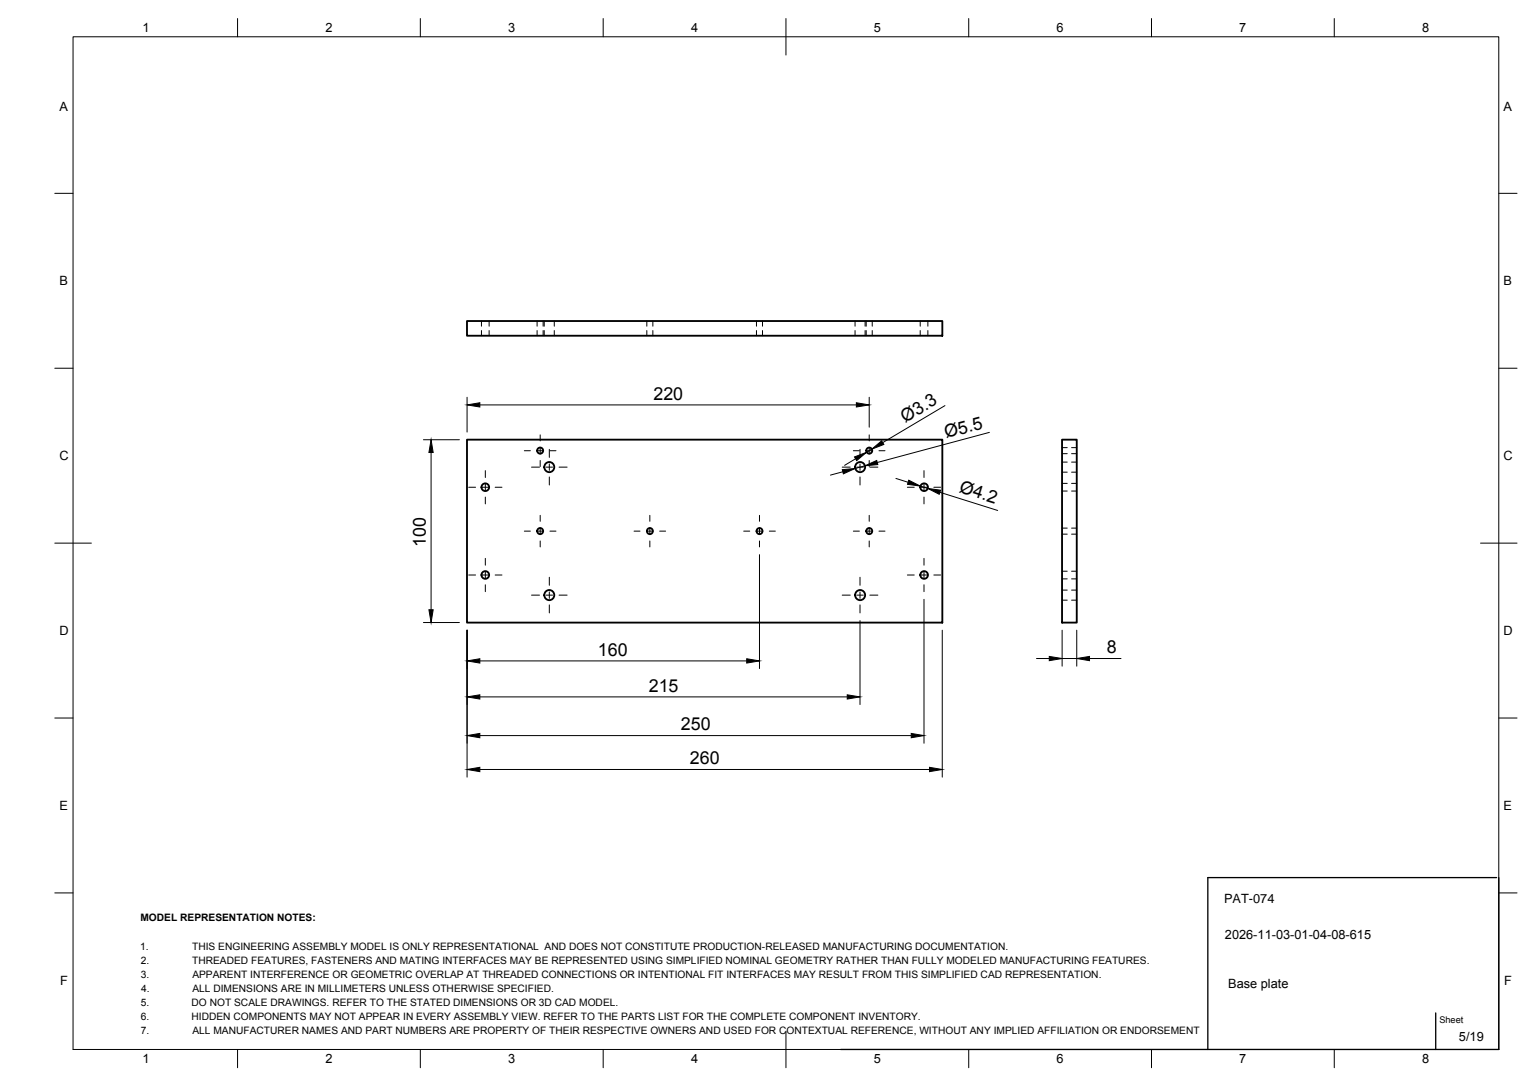
ISO-10303-21;
HEADER;
/* Generated by software containing ST-Developer
 * from STEP Tools, Inc. (www.steptools.com) 
 */

FILE_DESCRIPTION(
/* description */ ('Manual rail carriage with stops'),
/* implementation_level */ '2;1');

FILE_NAME(
/* name */ 'Base plate.step',
/* time_stamp */ '2026-10-27T18:54:27-07:00',
/* author */ (''),
/* organization */ (''),
/* preprocessor_version */ 'ST-DEVELOPER v20.2',
/* originating_system */ 'Autodesk Translation Framework v15.17.0.0',
/* authorisation */ '');

FILE_SCHEMA (('AUTOMOTIVE_DESIGN { 1 0 10303 214 3 1 1 }'));
ENDSEC;

DATA;
#10=MECHANICAL_DESIGN_GEOMETRIC_PRESENTATION_REPRESENTATION('',(#273),#8499);
#237=SHAPE_REPRESENTATION_RELATIONSHIP('SRR','None',#8600,#255);
#255=ADVANCED_BREP_SHAPE_REPRESENTATION('',(#291),#8479);
#273=STYLED_ITEM('',(#8767),#291);
#291=MANIFOLD_SOLID_BREP('Body1',#4941);
#305=FACE_BOUND('',#861,.T.);
#306=FACE_BOUND('',#862,.T.);
#307=FACE_BOUND('',#863,.T.);
#308=FACE_BOUND('',#864,.T.);
#309=FACE_BOUND('',#865,.T.);
#310=FACE_BOUND('',#866,.T.);
#311=FACE_BOUND('',#867,.T.);
#312=FACE_BOUND('',#868,.T.);
#313=FACE_BOUND('',#869,.T.);
#314=FACE_BOUND('',#870,.T.);
#315=FACE_BOUND('',#871,.T.);
#316=FACE_BOUND('',#872,.T.);
#317=FACE_BOUND('',#873,.T.);
#318=FACE_BOUND('',#874,.T.);
#319=FACE_BOUND('',#876,.T.);
#320=FACE_BOUND('',#877,.T.);
#321=FACE_BOUND('',#878,.T.);
#322=FACE_BOUND('',#879,.T.);
#323=FACE_BOUND('',#880,.T.);
#324=FACE_BOUND('',#881,.T.);
#325=FACE_BOUND('',#882,.T.);
#326=FACE_BOUND('',#883,.T.);
#327=FACE_BOUND('',#884,.T.);
#328=FACE_BOUND('',#885,.T.);
#329=FACE_BOUND('',#886,.T.);
#330=FACE_BOUND('',#887,.T.);
#331=FACE_BOUND('',#888,.T.);
#332=FACE_BOUND('',#889,.T.);
#380=PLANE('',#5207);
#381=PLANE('',#5208);
#382=PLANE('',#5209);
#383=PLANE('',#5210);
#384=PLANE('',#5211);
#385=PLANE('',#5212);
#577=FACE_OUTER_BOUND('',#842,.T.);
#578=FACE_OUTER_BOUND('',#843,.T.);
#579=FACE_OUTER_BOUND('',#844,.T.);
#580=FACE_OUTER_BOUND('',#845,.T.);
#581=FACE_OUTER_BOUND('',#846,.T.);
#582=FACE_OUTER_BOUND('',#847,.T.);
#583=FACE_OUTER_BOUND('',#848,.T.);
#584=FACE_OUTER_BOUND('',#849,.T.);
#585=FACE_OUTER_BOUND('',#850,.T.);
#586=FACE_OUTER_BOUND('',#851,.T.);
#587=FACE_OUTER_BOUND('',#852,.T.);
#588=FACE_OUTER_BOUND('',#853,.T.);
#589=FACE_OUTER_BOUND('',#854,.T.);
#590=FACE_OUTER_BOUND('',#855,.T.);
#591=FACE_OUTER_BOUND('',#856,.T.);
#592=FACE_OUTER_BOUND('',#857,.T.);
#593=FACE_OUTER_BOUND('',#858,.T.);
#594=FACE_OUTER_BOUND('',#859,.T.);
#595=FACE_OUTER_BOUND('',#860,.T.);
#596=FACE_OUTER_BOUND('',#875,.T.);
#842=EDGE_LOOP('',(#3360,#3361,#3362,#3363));
#843=EDGE_LOOP('',(#3364,#3365,#3366,#3367));
#844=EDGE_LOOP('',(#3368,#3369,#3370,#3371));
#845=EDGE_LOOP('',(#3372,#3373,#3374,#3375));
#846=EDGE_LOOP('',(#3376,#3377,#3378,#3379));
#847=EDGE_LOOP('',(#3380,#3381,#3382,#3383));
#848=EDGE_LOOP('',(#3384,#3385,#3386,#3387));
#849=EDGE_LOOP('',(#3388,#3389,#3390,#3391));
#850=EDGE_LOOP('',(#3392,#3393,#3394,#3395));
#851=EDGE_LOOP('',(#3396,#3397,#3398,#3399));
#852=EDGE_LOOP('',(#3400,#3401,#3402,#3403));
#853=EDGE_LOOP('',(#3404,#3405,#3406,#3407));
#854=EDGE_LOOP('',(#3408,#3409,#3410,#3411));
#855=EDGE_LOOP('',(#3412,#3413,#3414,#3415));
#856=EDGE_LOOP('',(#3416,#3417,#3418,#3419));
#857=EDGE_LOOP('',(#3420,#3421,#3422,#3423));
#858=EDGE_LOOP('',(#3424,#3425,#3426,#3427));
#859=EDGE_LOOP('',(#3428,#3429,#3430,#3431));
#860=EDGE_LOOP('',(#3432,#3433,#3434,#3435));
#861=EDGE_LOOP('',(#3436));
#862=EDGE_LOOP('',(#3437));
#863=EDGE_LOOP('',(#3438));
#864=EDGE_LOOP('',(#3439));
#865=EDGE_LOOP('',(#3440));
#866=EDGE_LOOP('',(#3441));
#867=EDGE_LOOP('',(#3442));
#868=EDGE_LOOP('',(#3443));
#869=EDGE_LOOP('',(#3444));
#870=EDGE_LOOP('',(#3445));
#871=EDGE_LOOP('',(#3446));
#872=EDGE_LOOP('',(#3447));
#873=EDGE_LOOP('',(#3448));
#874=EDGE_LOOP('',(#3449));
#875=EDGE_LOOP('',(#3450,#3451,#3452,#3453));
#876=EDGE_LOOP('',(#3454));
#877=EDGE_LOOP('',(#3455));
#878=EDGE_LOOP('',(#3456));
#879=EDGE_LOOP('',(#3457));
#880=EDGE_LOOP('',(#3458));
#881=EDGE_LOOP('',(#3459));
#882=EDGE_LOOP('',(#3460));
#883=EDGE_LOOP('',(#3461));
#884=EDGE_LOOP('',(#3462));
#885=EDGE_LOOP('',(#3463));
#886=EDGE_LOOP('',(#3464));
#887=EDGE_LOOP('',(#3465));
#888=EDGE_LOOP('',(#3466));
#889=EDGE_LOOP('',(#3467));
#1182=LINE('',#7076,#1682);
#1183=LINE('',#7082,#1683);
#1184=LINE('',#7088,#1684);
#1185=LINE('',#7094,#1685);
#1186=LINE('',#7100,#1686);
#1187=LINE('',#7106,#1687);
#1188=LINE('',#7112,#1688);
#1189=LINE('',#7118,#1689);
#1190=LINE('',#7124,#1690);
#1191=LINE('',#7130,#1691);
#1192=LINE('',#7136,#1692);
#1193=LINE('',#7142,#1693);
#1194=LINE('',#7148,#1694);
#1195=LINE('',#7154,#1695);
#1196=LINE('',#7159,#1696);
#1197=LINE('',#7161,#1697);
#1198=LINE('',#7163,#1698);
#1199=LINE('',#7164,#1699);
#1200=LINE('',#7167,#1700);
#1201=LINE('',#7169,#1701);
#1202=LINE('',#7170,#1702);
#1203=LINE('',#7173,#1703);
#1204=LINE('',#7175,#1704);
#1205=LINE('',#7176,#1705);
#1206=LINE('',#7178,#1706);
#1207=LINE('',#7179,#1707);
#1682=VECTOR('',#5641,0.165);
#1683=VECTOR('',#5648,0.164999999999999);
#1684=VECTOR('',#5655,0.210000000000001);
#1685=VECTOR('',#5662,0.21);
#1686=VECTOR('',#5669,0.21);
#1687=VECTOR('',#5676,0.210000000000001);
#1688=VECTOR('',#5683,0.274999999999999);
#1689=VECTOR('',#5690,0.275);
#1690=VECTOR('',#5697,0.275);
#1691=VECTOR('',#5704,0.274999999999999);
#1692=VECTOR('',#5711,0.164999999999999);
#1693=VECTOR('',#5718,0.164999999999999);
#1694=VECTOR('',#5725,0.165);
#1695=VECTOR('',#5732,0.164999999999999);
#1696=VECTOR('',#5737,1.);
#1697=VECTOR('',#5738,1.);
#1698=VECTOR('',#5739,1.);
#1699=VECTOR('',#5740,1.);
#1700=VECTOR('',#5743,1.);
#1701=VECTOR('',#5744,1.);
#1702=VECTOR('',#5745,1.);
#1703=VECTOR('',#5748,1.);
#1704=VECTOR('',#5749,1.);
#1705=VECTOR('',#5750,1.);
#1706=VECTOR('',#5753,1.);
#1707=VECTOR('',#5754,1.);
#2182=CIRCLE('',#5166,0.165);
#2183=CIRCLE('',#5167,0.165);
#2184=CIRCLE('',#5169,0.164999999999999);
#2185=CIRCLE('',#5170,0.164999999999999);
#2186=CIRCLE('',#5172,0.210000000000001);
#2187=CIRCLE('',#5173,0.210000000000001);
#2188=CIRCLE('',#5175,0.21);
#2189=CIRCLE('',#5176,0.21);
#2190=CIRCLE('',#5178,0.21);
#2191=CIRCLE('',#5179,0.21);
#2192=CIRCLE('',#5181,0.210000000000001);
#2193=CIRCLE('',#5182,0.210000000000001);
#2194=CIRCLE('',#5184,0.274999999999999);
#2195=CIRCLE('',#5185,0.274999999999999);
#2196=CIRCLE('',#5187,0.275);
#2197=CIRCLE('',#5188,0.275);
#2198=CIRCLE('',#5190,0.275);
#2199=CIRCLE('',#5191,0.275);
#2200=CIRCLE('',#5193,0.274999999999999);
#2201=CIRCLE('',#5194,0.274999999999999);
#2202=CIRCLE('',#5196,0.164999999999999);
#2203=CIRCLE('',#5197,0.164999999999999);
#2204=CIRCLE('',#5199,0.164999999999999);
#2205=CIRCLE('',#5200,0.164999999999999);
#2206=CIRCLE('',#5202,0.165);
#2207=CIRCLE('',#5203,0.165);
#2208=CIRCLE('',#5205,0.164999999999999);
#2209=CIRCLE('',#5206,0.164999999999999);
#2312=VERTEX_POINT('',#7073);
#2313=VERTEX_POINT('',#7075);
#2314=VERTEX_POINT('',#7079);
#2315=VERTEX_POINT('',#7081);
#2316=VERTEX_POINT('',#7085);
#2317=VERTEX_POINT('',#7087);
#2318=VERTEX_POINT('',#7091);
#2319=VERTEX_POINT('',#7093);
#2320=VERTEX_POINT('',#7097);
#2321=VERTEX_POINT('',#7099);
#2322=VERTEX_POINT('',#7103);
#2323=VERTEX_POINT('',#7105);
#2324=VERTEX_POINT('',#7109);
#2325=VERTEX_POINT('',#7111);
#2326=VERTEX_POINT('',#7115);
#2327=VERTEX_POINT('',#7117);
#2328=VERTEX_POINT('',#7121);
#2329=VERTEX_POINT('',#7123);
#2330=VERTEX_POINT('',#7127);
#2331=VERTEX_POINT('',#7129);
#2332=VERTEX_POINT('',#7133);
#2333=VERTEX_POINT('',#7135);
#2334=VERTEX_POINT('',#7139);
#2335=VERTEX_POINT('',#7141);
#2336=VERTEX_POINT('',#7145);
#2337=VERTEX_POINT('',#7147);
#2338=VERTEX_POINT('',#7151);
#2339=VERTEX_POINT('',#7153);
#2340=VERTEX_POINT('',#7157);
#2341=VERTEX_POINT('',#7158);
#2342=VERTEX_POINT('',#7160);
#2343=VERTEX_POINT('',#7162);
#2344=VERTEX_POINT('',#7166);
#2345=VERTEX_POINT('',#7168);
#2346=VERTEX_POINT('',#7172);
#2347=VERTEX_POINT('',#7174);
#2728=EDGE_CURVE('',#2312,#2312,#2182,.T.);
#2729=EDGE_CURVE('',#2312,#2313,#1182,.T.);
#2730=EDGE_CURVE('',#2313,#2313,#2183,.T.);
#2731=EDGE_CURVE('',#2314,#2314,#2184,.T.);
#2732=EDGE_CURVE('',#2314,#2315,#1183,.T.);
#2733=EDGE_CURVE('',#2315,#2315,#2185,.T.);
#2734=EDGE_CURVE('',#2316,#2316,#2186,.T.);
#2735=EDGE_CURVE('',#2316,#2317,#1184,.T.);
#2736=EDGE_CURVE('',#2317,#2317,#2187,.T.);
#2737=EDGE_CURVE('',#2318,#2318,#2188,.T.);
#2738=EDGE_CURVE('',#2318,#2319,#1185,.T.);
#2739=EDGE_CURVE('',#2319,#2319,#2189,.T.);
#2740=EDGE_CURVE('',#2320,#2320,#2190,.T.);
#2741=EDGE_CURVE('',#2320,#2321,#1186,.T.);
#2742=EDGE_CURVE('',#2321,#2321,#2191,.T.);
#2743=EDGE_CURVE('',#2322,#2322,#2192,.T.);
#2744=EDGE_CURVE('',#2322,#2323,#1187,.T.);
#2745=EDGE_CURVE('',#2323,#2323,#2193,.T.);
#2746=EDGE_CURVE('',#2324,#2324,#2194,.T.);
#2747=EDGE_CURVE('',#2324,#2325,#1188,.T.);
#2748=EDGE_CURVE('',#2325,#2325,#2195,.T.);
#2749=EDGE_CURVE('',#2326,#2326,#2196,.T.);
#2750=EDGE_CURVE('',#2326,#2327,#1189,.T.);
#2751=EDGE_CURVE('',#2327,#2327,#2197,.T.);
#2752=EDGE_CURVE('',#2328,#2328,#2198,.T.);
#2753=EDGE_CURVE('',#2328,#2329,#1190,.T.);
#2754=EDGE_CURVE('',#2329,#2329,#2199,.T.);
#2755=EDGE_CURVE('',#2330,#2330,#2200,.T.);
#2756=EDGE_CURVE('',#2330,#2331,#1191,.T.);
#2757=EDGE_CURVE('',#2331,#2331,#2201,.T.);
#2758=EDGE_CURVE('',#2332,#2332,#2202,.T.);
#2759=EDGE_CURVE('',#2332,#2333,#1192,.T.);
#2760=EDGE_CURVE('',#2333,#2333,#2203,.T.);
#2761=EDGE_CURVE('',#2334,#2334,#2204,.T.);
#2762=EDGE_CURVE('',#2334,#2335,#1193,.T.);
#2763=EDGE_CURVE('',#2335,#2335,#2205,.T.);
#2764=EDGE_CURVE('',#2336,#2336,#2206,.T.);
#2765=EDGE_CURVE('',#2336,#2337,#1194,.T.);
#2766=EDGE_CURVE('',#2337,#2337,#2207,.T.);
#2767=EDGE_CURVE('',#2338,#2338,#2208,.T.);
#2768=EDGE_CURVE('',#2338,#2339,#1195,.T.);
#2769=EDGE_CURVE('',#2339,#2339,#2209,.T.);
#2770=EDGE_CURVE('',#2340,#2341,#1196,.T.);
#2771=EDGE_CURVE('',#2341,#2342,#1197,.T.);
#2772=EDGE_CURVE('',#2343,#2342,#1198,.T.);
#2773=EDGE_CURVE('',#2340,#2343,#1199,.T.);
#2774=EDGE_CURVE('',#2344,#2340,#1200,.T.);
#2775=EDGE_CURVE('',#2345,#2343,#1201,.T.);
#2776=EDGE_CURVE('',#2344,#2345,#1202,.T.);
#2777=EDGE_CURVE('',#2346,#2344,#1203,.T.);
#2778=EDGE_CURVE('',#2347,#2345,#1204,.T.);
#2779=EDGE_CURVE('',#2346,#2347,#1205,.T.);
#2780=EDGE_CURVE('',#2341,#2346,#1206,.T.);
#2781=EDGE_CURVE('',#2342,#2347,#1207,.T.);
#3360=ORIENTED_EDGE('',*,*,#2728,.F.);
#3361=ORIENTED_EDGE('',*,*,#2729,.T.);
#3362=ORIENTED_EDGE('',*,*,#2730,.F.);
#3363=ORIENTED_EDGE('',*,*,#2729,.F.);
#3364=ORIENTED_EDGE('',*,*,#2731,.F.);
#3365=ORIENTED_EDGE('',*,*,#2732,.T.);
#3366=ORIENTED_EDGE('',*,*,#2733,.F.);
#3367=ORIENTED_EDGE('',*,*,#2732,.F.);
#3368=ORIENTED_EDGE('',*,*,#2734,.F.);
#3369=ORIENTED_EDGE('',*,*,#2735,.T.);
#3370=ORIENTED_EDGE('',*,*,#2736,.F.);
#3371=ORIENTED_EDGE('',*,*,#2735,.F.);
#3372=ORIENTED_EDGE('',*,*,#2737,.F.);
#3373=ORIENTED_EDGE('',*,*,#2738,.T.);
#3374=ORIENTED_EDGE('',*,*,#2739,.F.);
#3375=ORIENTED_EDGE('',*,*,#2738,.F.);
#3376=ORIENTED_EDGE('',*,*,#2740,.F.);
#3377=ORIENTED_EDGE('',*,*,#2741,.T.);
#3378=ORIENTED_EDGE('',*,*,#2742,.F.);
#3379=ORIENTED_EDGE('',*,*,#2741,.F.);
#3380=ORIENTED_EDGE('',*,*,#2743,.F.);
#3381=ORIENTED_EDGE('',*,*,#2744,.T.);
#3382=ORIENTED_EDGE('',*,*,#2745,.F.);
#3383=ORIENTED_EDGE('',*,*,#2744,.F.);
#3384=ORIENTED_EDGE('',*,*,#2746,.F.);
#3385=ORIENTED_EDGE('',*,*,#2747,.T.);
#3386=ORIENTED_EDGE('',*,*,#2748,.F.);
#3387=ORIENTED_EDGE('',*,*,#2747,.F.);
#3388=ORIENTED_EDGE('',*,*,#2749,.F.);
#3389=ORIENTED_EDGE('',*,*,#2750,.T.);
#3390=ORIENTED_EDGE('',*,*,#2751,.F.);
#3391=ORIENTED_EDGE('',*,*,#2750,.F.);
#3392=ORIENTED_EDGE('',*,*,#2752,.F.);
#3393=ORIENTED_EDGE('',*,*,#2753,.T.);
#3394=ORIENTED_EDGE('',*,*,#2754,.F.);
#3395=ORIENTED_EDGE('',*,*,#2753,.F.);
#3396=ORIENTED_EDGE('',*,*,#2755,.F.);
#3397=ORIENTED_EDGE('',*,*,#2756,.T.);
#3398=ORIENTED_EDGE('',*,*,#2757,.F.);
#3399=ORIENTED_EDGE('',*,*,#2756,.F.);
#3400=ORIENTED_EDGE('',*,*,#2758,.F.);
#3401=ORIENTED_EDGE('',*,*,#2759,.T.);
#3402=ORIENTED_EDGE('',*,*,#2760,.F.);
#3403=ORIENTED_EDGE('',*,*,#2759,.F.);
#3404=ORIENTED_EDGE('',*,*,#2761,.F.);
#3405=ORIENTED_EDGE('',*,*,#2762,.T.);
#3406=ORIENTED_EDGE('',*,*,#2763,.F.);
#3407=ORIENTED_EDGE('',*,*,#2762,.F.);
#3408=ORIENTED_EDGE('',*,*,#2764,.F.);
#3409=ORIENTED_EDGE('',*,*,#2765,.T.);
#3410=ORIENTED_EDGE('',*,*,#2766,.F.);
#3411=ORIENTED_EDGE('',*,*,#2765,.F.);
#3412=ORIENTED_EDGE('',*,*,#2767,.F.);
#3413=ORIENTED_EDGE('',*,*,#2768,.T.);
#3414=ORIENTED_EDGE('',*,*,#2769,.F.);
#3415=ORIENTED_EDGE('',*,*,#2768,.F.);
#3416=ORIENTED_EDGE('',*,*,#2770,.T.);
#3417=ORIENTED_EDGE('',*,*,#2771,.T.);
#3418=ORIENTED_EDGE('',*,*,#2772,.F.);
#3419=ORIENTED_EDGE('',*,*,#2773,.F.);
#3420=ORIENTED_EDGE('',*,*,#2774,.T.);
#3421=ORIENTED_EDGE('',*,*,#2773,.T.);
#3422=ORIENTED_EDGE('',*,*,#2775,.F.);
#3423=ORIENTED_EDGE('',*,*,#2776,.F.);
#3424=ORIENTED_EDGE('',*,*,#2777,.T.);
#3425=ORIENTED_EDGE('',*,*,#2776,.T.);
#3426=ORIENTED_EDGE('',*,*,#2778,.F.);
#3427=ORIENTED_EDGE('',*,*,#2779,.F.);
#3428=ORIENTED_EDGE('',*,*,#2780,.T.);
#3429=ORIENTED_EDGE('',*,*,#2779,.T.);
#3430=ORIENTED_EDGE('',*,*,#2781,.F.);
#3431=ORIENTED_EDGE('',*,*,#2771,.F.);
#3432=ORIENTED_EDGE('',*,*,#2781,.T.);
#3433=ORIENTED_EDGE('',*,*,#2778,.T.);
#3434=ORIENTED_EDGE('',*,*,#2775,.T.);
#3435=ORIENTED_EDGE('',*,*,#2772,.T.);
#3436=ORIENTED_EDGE('',*,*,#2736,.T.);
#3437=ORIENTED_EDGE('',*,*,#2739,.T.);
#3438=ORIENTED_EDGE('',*,*,#2742,.T.);
#3439=ORIENTED_EDGE('',*,*,#2745,.T.);
#3440=ORIENTED_EDGE('',*,*,#2769,.T.);
#3441=ORIENTED_EDGE('',*,*,#2766,.T.);
#3442=ORIENTED_EDGE('',*,*,#2763,.T.);
#3443=ORIENTED_EDGE('',*,*,#2760,.T.);
#3444=ORIENTED_EDGE('',*,*,#2757,.T.);
#3445=ORIENTED_EDGE('',*,*,#2754,.T.);
#3446=ORIENTED_EDGE('',*,*,#2751,.T.);
#3447=ORIENTED_EDGE('',*,*,#2748,.T.);
#3448=ORIENTED_EDGE('',*,*,#2733,.T.);
#3449=ORIENTED_EDGE('',*,*,#2730,.T.);
#3450=ORIENTED_EDGE('',*,*,#2780,.F.);
#3451=ORIENTED_EDGE('',*,*,#2770,.F.);
#3452=ORIENTED_EDGE('',*,*,#2774,.F.);
#3453=ORIENTED_EDGE('',*,*,#2777,.F.);
#3454=ORIENTED_EDGE('',*,*,#2734,.T.);
#3455=ORIENTED_EDGE('',*,*,#2737,.T.);
#3456=ORIENTED_EDGE('',*,*,#2740,.T.);
#3457=ORIENTED_EDGE('',*,*,#2743,.T.);
#3458=ORIENTED_EDGE('',*,*,#2767,.T.);
#3459=ORIENTED_EDGE('',*,*,#2764,.T.);
#3460=ORIENTED_EDGE('',*,*,#2761,.T.);
#3461=ORIENTED_EDGE('',*,*,#2758,.T.);
#3462=ORIENTED_EDGE('',*,*,#2755,.T.);
#3463=ORIENTED_EDGE('',*,*,#2752,.T.);
#3464=ORIENTED_EDGE('',*,*,#2749,.T.);
#3465=ORIENTED_EDGE('',*,*,#2746,.T.);
#3466=ORIENTED_EDGE('',*,*,#2731,.T.);
#3467=ORIENTED_EDGE('',*,*,#2728,.T.);
#4624=CYLINDRICAL_SURFACE('',#5165,0.165);
#4625=CYLINDRICAL_SURFACE('',#5168,0.164999999999999);
#4626=CYLINDRICAL_SURFACE('',#5171,0.210000000000001);
#4627=CYLINDRICAL_SURFACE('',#5174,0.21);
#4628=CYLINDRICAL_SURFACE('',#5177,0.21);
#4629=CYLINDRICAL_SURFACE('',#5180,0.210000000000001);
#4630=CYLINDRICAL_SURFACE('',#5183,0.274999999999999);
#4631=CYLINDRICAL_SURFACE('',#5186,0.275);
#4632=CYLINDRICAL_SURFACE('',#5189,0.275);
#4633=CYLINDRICAL_SURFACE('',#5192,0.274999999999999);
#4634=CYLINDRICAL_SURFACE('',#5195,0.164999999999999);
#4635=CYLINDRICAL_SURFACE('',#5198,0.164999999999999);
#4636=CYLINDRICAL_SURFACE('',#5201,0.165);
#4637=CYLINDRICAL_SURFACE('',#5204,0.164999999999999);
#4676=ADVANCED_FACE('',(#577),#4624,.F.);
#4677=ADVANCED_FACE('',(#578),#4625,.F.);
#4678=ADVANCED_FACE('',(#579),#4626,.F.);
#4679=ADVANCED_FACE('',(#580),#4627,.F.);
#4680=ADVANCED_FACE('',(#581),#4628,.F.);
#4681=ADVANCED_FACE('',(#582),#4629,.F.);
#4682=ADVANCED_FACE('',(#583),#4630,.F.);
#4683=ADVANCED_FACE('',(#584),#4631,.F.);
#4684=ADVANCED_FACE('',(#585),#4632,.F.);
#4685=ADVANCED_FACE('',(#586),#4633,.F.);
#4686=ADVANCED_FACE('',(#587),#4634,.F.);
#4687=ADVANCED_FACE('',(#588),#4635,.F.);
#4688=ADVANCED_FACE('',(#589),#4636,.F.);
#4689=ADVANCED_FACE('',(#590),#4637,.F.);
#4690=ADVANCED_FACE('',(#591),#380,.T.);
#4691=ADVANCED_FACE('',(#592),#381,.T.);
#4692=ADVANCED_FACE('',(#593),#382,.T.);
#4693=ADVANCED_FACE('',(#594),#383,.T.);
#4694=ADVANCED_FACE('',(#595,#305,#306,#307,#308,#309,#310,#311,#312,#313,
#314,#315,#316,#317,#318),#384,.T.);
#4695=ADVANCED_FACE('',(#596,#319,#320,#321,#322,#323,#324,#325,#326,#327,
#328,#329,#330,#331,#332),#385,.F.);
#4941=CLOSED_SHELL('',(#4676,#4677,#4678,#4679,#4680,#4681,#4682,#4683,
#4684,#4685,#4686,#4687,#4688,#4689,#4690,#4691,#4692,#4693,#4694,#4695));
#5164=AXIS2_PLACEMENT_3D('',#7071,#5635,#5636);
#5165=AXIS2_PLACEMENT_3D('',#7072,#5637,#5638);
#5166=AXIS2_PLACEMENT_3D('',#7074,#5639,#5640);
#5167=AXIS2_PLACEMENT_3D('',#7077,#5642,#5643);
#5168=AXIS2_PLACEMENT_3D('',#7078,#5644,#5645);
#5169=AXIS2_PLACEMENT_3D('',#7080,#5646,#5647);
#5170=AXIS2_PLACEMENT_3D('',#7083,#5649,#5650);
#5171=AXIS2_PLACEMENT_3D('',#7084,#5651,#5652);
#5172=AXIS2_PLACEMENT_3D('',#7086,#5653,#5654);
#5173=AXIS2_PLACEMENT_3D('',#7089,#5656,#5657);
#5174=AXIS2_PLACEMENT_3D('',#7090,#5658,#5659);
#5175=AXIS2_PLACEMENT_3D('',#7092,#5660,#5661);
#5176=AXIS2_PLACEMENT_3D('',#7095,#5663,#5664);
#5177=AXIS2_PLACEMENT_3D('',#7096,#5665,#5666);
#5178=AXIS2_PLACEMENT_3D('',#7098,#5667,#5668);
#5179=AXIS2_PLACEMENT_3D('',#7101,#5670,#5671);
#5180=AXIS2_PLACEMENT_3D('',#7102,#5672,#5673);
#5181=AXIS2_PLACEMENT_3D('',#7104,#5674,#5675);
#5182=AXIS2_PLACEMENT_3D('',#7107,#5677,#5678);
#5183=AXIS2_PLACEMENT_3D('',#7108,#5679,#5680);
#5184=AXIS2_PLACEMENT_3D('',#7110,#5681,#5682);
#5185=AXIS2_PLACEMENT_3D('',#7113,#5684,#5685);
#5186=AXIS2_PLACEMENT_3D('',#7114,#5686,#5687);
#5187=AXIS2_PLACEMENT_3D('',#7116,#5688,#5689);
#5188=AXIS2_PLACEMENT_3D('',#7119,#5691,#5692);
#5189=AXIS2_PLACEMENT_3D('',#7120,#5693,#5694);
#5190=AXIS2_PLACEMENT_3D('',#7122,#5695,#5696);
#5191=AXIS2_PLACEMENT_3D('',#7125,#5698,#5699);
#5192=AXIS2_PLACEMENT_3D('',#7126,#5700,#5701);
#5193=AXIS2_PLACEMENT_3D('',#7128,#5702,#5703);
#5194=AXIS2_PLACEMENT_3D('',#7131,#5705,#5706);
#5195=AXIS2_PLACEMENT_3D('',#7132,#5707,#5708);
#5196=AXIS2_PLACEMENT_3D('',#7134,#5709,#5710);
#5197=AXIS2_PLACEMENT_3D('',#7137,#5712,#5713);
#5198=AXIS2_PLACEMENT_3D('',#7138,#5714,#5715);
#5199=AXIS2_PLACEMENT_3D('',#7140,#5716,#5717);
#5200=AXIS2_PLACEMENT_3D('',#7143,#5719,#5720);
#5201=AXIS2_PLACEMENT_3D('',#7144,#5721,#5722);
#5202=AXIS2_PLACEMENT_3D('',#7146,#5723,#5724);
#5203=AXIS2_PLACEMENT_3D('',#7149,#5726,#5727);
#5204=AXIS2_PLACEMENT_3D('',#7150,#5728,#5729);
#5205=AXIS2_PLACEMENT_3D('',#7152,#5730,#5731);
#5206=AXIS2_PLACEMENT_3D('',#7155,#5733,#5734);
#5207=AXIS2_PLACEMENT_3D('',#7156,#5735,#5736);
#5208=AXIS2_PLACEMENT_3D('',#7165,#5741,#5742);
#5209=AXIS2_PLACEMENT_3D('',#7171,#5746,#5747);
#5210=AXIS2_PLACEMENT_3D('',#7177,#5751,#5752);
#5211=AXIS2_PLACEMENT_3D('',#7180,#5755,#5756);
#5212=AXIS2_PLACEMENT_3D('',#7181,#5757,#5758);
#5635=DIRECTION('axis',(0.,0.,1.));
#5636=DIRECTION('refdir',(1.,0.,0.));
#5637=DIRECTION('center_axis',(0.,0.,1.));
#5638=DIRECTION('ref_axis',(1.,0.,0.));
#5639=DIRECTION('center_axis',(0.,0.,1.));
#5640=DIRECTION('ref_axis',(1.,0.,0.));
#5641=DIRECTION('',(0.,0.,1.));
#5642=DIRECTION('center_axis',(0.,0.,-1.));
#5643=DIRECTION('ref_axis',(1.,0.,0.));
#5644=DIRECTION('center_axis',(0.,0.,1.));
#5645=DIRECTION('ref_axis',(1.,0.,0.));
#5646=DIRECTION('center_axis',(0.,0.,1.));
#5647=DIRECTION('ref_axis',(1.,0.,0.));
#5648=DIRECTION('',(0.,0.,1.));
#5649=DIRECTION('center_axis',(0.,0.,-1.));
#5650=DIRECTION('ref_axis',(1.,0.,0.));
#5651=DIRECTION('center_axis',(0.,0.,1.));
#5652=DIRECTION('ref_axis',(1.,0.,0.));
#5653=DIRECTION('center_axis',(0.,0.,1.));
#5654=DIRECTION('ref_axis',(1.,0.,0.));
#5655=DIRECTION('',(0.,0.,1.));
#5656=DIRECTION('center_axis',(0.,0.,-1.));
#5657=DIRECTION('ref_axis',(1.,0.,0.));
#5658=DIRECTION('center_axis',(0.,0.,1.));
#5659=DIRECTION('ref_axis',(1.,0.,0.));
#5660=DIRECTION('center_axis',(0.,0.,1.));
#5661=DIRECTION('ref_axis',(1.,0.,0.));
#5662=DIRECTION('',(0.,0.,1.));
#5663=DIRECTION('center_axis',(0.,0.,-1.));
#5664=DIRECTION('ref_axis',(1.,0.,0.));
#5665=DIRECTION('center_axis',(0.,0.,1.));
#5666=DIRECTION('ref_axis',(1.,0.,0.));
#5667=DIRECTION('center_axis',(0.,0.,1.));
#5668=DIRECTION('ref_axis',(1.,0.,0.));
#5669=DIRECTION('',(0.,0.,1.));
#5670=DIRECTION('center_axis',(0.,0.,-1.));
#5671=DIRECTION('ref_axis',(1.,0.,0.));
#5672=DIRECTION('center_axis',(0.,0.,1.));
#5673=DIRECTION('ref_axis',(1.,0.,0.));
#5674=DIRECTION('center_axis',(0.,0.,1.));
#5675=DIRECTION('ref_axis',(1.,0.,0.));
#5676=DIRECTION('',(0.,0.,1.));
#5677=DIRECTION('center_axis',(0.,0.,-1.));
#5678=DIRECTION('ref_axis',(1.,0.,0.));
#5679=DIRECTION('center_axis',(0.,0.,1.));
#5680=DIRECTION('ref_axis',(1.,0.,0.));
#5681=DIRECTION('center_axis',(0.,0.,1.));
#5682=DIRECTION('ref_axis',(1.,0.,0.));
#5683=DIRECTION('',(0.,0.,1.));
#5684=DIRECTION('center_axis',(0.,0.,-1.));
#5685=DIRECTION('ref_axis',(1.,0.,0.));
#5686=DIRECTION('center_axis',(0.,0.,1.));
#5687=DIRECTION('ref_axis',(1.,0.,0.));
#5688=DIRECTION('center_axis',(0.,0.,1.));
#5689=DIRECTION('ref_axis',(1.,0.,0.));
#5690=DIRECTION('',(0.,0.,1.));
#5691=DIRECTION('center_axis',(0.,0.,-1.));
#5692=DIRECTION('ref_axis',(1.,0.,0.));
#5693=DIRECTION('center_axis',(0.,0.,1.));
#5694=DIRECTION('ref_axis',(1.,0.,0.));
#5695=DIRECTION('center_axis',(0.,0.,1.));
#5696=DIRECTION('ref_axis',(1.,0.,0.));
#5697=DIRECTION('',(0.,0.,1.));
#5698=DIRECTION('center_axis',(0.,0.,-1.));
#5699=DIRECTION('ref_axis',(1.,0.,0.));
#5700=DIRECTION('center_axis',(0.,0.,1.));
#5701=DIRECTION('ref_axis',(1.,0.,0.));
#5702=DIRECTION('center_axis',(0.,0.,1.));
#5703=DIRECTION('ref_axis',(1.,0.,0.));
#5704=DIRECTION('',(0.,0.,1.));
#5705=DIRECTION('center_axis',(0.,0.,-1.));
#5706=DIRECTION('ref_axis',(1.,0.,0.));
#5707=DIRECTION('center_axis',(0.,0.,1.));
#5708=DIRECTION('ref_axis',(1.,0.,0.));
#5709=DIRECTION('center_axis',(0.,0.,1.));
#5710=DIRECTION('ref_axis',(1.,0.,0.));
#5711=DIRECTION('',(0.,0.,1.));
#5712=DIRECTION('center_axis',(0.,0.,-1.));
#5713=DIRECTION('ref_axis',(1.,0.,0.));
#5714=DIRECTION('center_axis',(0.,0.,1.));
#5715=DIRECTION('ref_axis',(1.,0.,0.));
#5716=DIRECTION('center_axis',(0.,0.,1.));
#5717=DIRECTION('ref_axis',(1.,0.,0.));
#5718=DIRECTION('',(0.,0.,1.));
#5719=DIRECTION('center_axis',(0.,0.,-1.));
#5720=DIRECTION('ref_axis',(1.,0.,0.));
#5721=DIRECTION('center_axis',(0.,0.,1.));
#5722=DIRECTION('ref_axis',(1.,0.,0.));
#5723=DIRECTION('center_axis',(0.,0.,1.));
#5724=DIRECTION('ref_axis',(1.,0.,0.));
#5725=DIRECTION('',(0.,0.,1.));
#5726=DIRECTION('center_axis',(0.,0.,-1.));
#5727=DIRECTION('ref_axis',(1.,0.,0.));
#5728=DIRECTION('center_axis',(0.,0.,1.));
#5729=DIRECTION('ref_axis',(1.,0.,0.));
#5730=DIRECTION('center_axis',(0.,0.,1.));
#5731=DIRECTION('ref_axis',(1.,0.,0.));
#5732=DIRECTION('',(0.,0.,1.));
#5733=DIRECTION('center_axis',(0.,0.,-1.));
#5734=DIRECTION('ref_axis',(1.,0.,0.));
#5735=DIRECTION('center_axis',(0.,1.,0.));
#5736=DIRECTION('ref_axis',(-1.,0.,0.));
#5737=DIRECTION('',(-1.,0.,0.));
#5738=DIRECTION('',(0.,0.,1.));
#5739=DIRECTION('',(-1.,0.,0.));
#5740=DIRECTION('',(0.,0.,1.));
#5741=DIRECTION('center_axis',(1.,0.,0.));
#5742=DIRECTION('ref_axis',(0.,1.,0.));
#5743=DIRECTION('',(0.,1.,0.));
#5744=DIRECTION('',(0.,1.,0.));
#5745=DIRECTION('',(0.,0.,1.));
#5746=DIRECTION('center_axis',(0.,-1.,0.));
#5747=DIRECTION('ref_axis',(1.,0.,0.));
#5748=DIRECTION('',(1.,0.,0.));
#5749=DIRECTION('',(1.,0.,0.));
#5750=DIRECTION('',(0.,0.,1.));
#5751=DIRECTION('center_axis',(-1.,0.,0.));
#5752=DIRECTION('ref_axis',(0.,-1.,0.));
#5753=DIRECTION('',(0.,-1.,0.));
#5754=DIRECTION('',(0.,-1.,0.));
#5755=DIRECTION('center_axis',(0.,0.,1.));
#5756=DIRECTION('ref_axis',(1.,0.,0.));
#5757=DIRECTION('center_axis',(0.,0.,1.));
#5758=DIRECTION('ref_axis',(1.,0.,0.));
#7071=CARTESIAN_POINT('',(0.,0.,0.));
#7072=CARTESIAN_POINT('Origin',(2.,4.4,1.9));
#7073=CARTESIAN_POINT('',(1.835,4.4,2.));
#7074=CARTESIAN_POINT('Origin',(2.,4.4,2.));
#7075=CARTESIAN_POINT('',(1.835,4.4,2.8));
#7076=CARTESIAN_POINT('',(1.835,4.4,1.9));
#7077=CARTESIAN_POINT('Origin',(2.,4.4,2.8));
#7078=CARTESIAN_POINT('Origin',(20.,4.4,1.9));
#7079=CARTESIAN_POINT('',(19.835,4.4,2.));
#7080=CARTESIAN_POINT('Origin',(20.,4.4,2.));
#7081=CARTESIAN_POINT('',(19.835,4.4,2.8));
#7082=CARTESIAN_POINT('',(19.835,4.4,1.9));
#7083=CARTESIAN_POINT('Origin',(20.,4.4,2.8));
#7084=CARTESIAN_POINT('Origin',(23.,-2.4,1.9));
#7085=CARTESIAN_POINT('',(22.79,-2.4,2.));
#7086=CARTESIAN_POINT('Origin',(23.,-2.4,2.));
#7087=CARTESIAN_POINT('',(22.79,-2.4,2.8));
#7088=CARTESIAN_POINT('',(22.79,-2.4,1.9));
#7089=CARTESIAN_POINT('Origin',(23.,-2.4,2.8));
#7090=CARTESIAN_POINT('Origin',(-1.,2.4,1.9));
#7091=CARTESIAN_POINT('',(-1.21,2.4,2.));
#7092=CARTESIAN_POINT('Origin',(-1.,2.4,2.));
#7093=CARTESIAN_POINT('',(-1.21,2.4,2.8));
#7094=CARTESIAN_POINT('',(-1.21,2.4,1.9));
#7095=CARTESIAN_POINT('Origin',(-1.,2.4,2.8));
#7096=CARTESIAN_POINT('Origin',(-1.,-2.4,1.9));
#7097=CARTESIAN_POINT('',(-1.21,-2.4,2.));
#7098=CARTESIAN_POINT('Origin',(-1.,-2.4,2.));
#7099=CARTESIAN_POINT('',(-1.21,-2.4,2.8));
#7100=CARTESIAN_POINT('',(-1.21,-2.4,1.9));
#7101=CARTESIAN_POINT('Origin',(-1.,-2.4,2.8));
#7102=CARTESIAN_POINT('Origin',(23.,2.4,1.9));
#7103=CARTESIAN_POINT('',(22.79,2.4,2.));
#7104=CARTESIAN_POINT('Origin',(23.,2.4,2.));
#7105=CARTESIAN_POINT('',(22.79,2.4,2.8));
#7106=CARTESIAN_POINT('',(22.79,2.4,1.9));
#7107=CARTESIAN_POINT('Origin',(23.,2.4,2.8));
#7108=CARTESIAN_POINT('Origin',(19.5,-3.5,1.9));
#7109=CARTESIAN_POINT('',(19.225,-3.5,2.));
#7110=CARTESIAN_POINT('Origin',(19.5,-3.5,2.));
#7111=CARTESIAN_POINT('',(19.225,-3.5,2.8));
#7112=CARTESIAN_POINT('',(19.225,-3.5,1.9));
#7113=CARTESIAN_POINT('Origin',(19.5,-3.5,2.8));
#7114=CARTESIAN_POINT('Origin',(2.5,3.5,1.9));
#7115=CARTESIAN_POINT('',(2.225,3.5,2.));
#7116=CARTESIAN_POINT('Origin',(2.5,3.5,2.));
#7117=CARTESIAN_POINT('',(2.225,3.5,2.8));
#7118=CARTESIAN_POINT('',(2.225,3.5,1.9));
#7119=CARTESIAN_POINT('Origin',(2.5,3.5,2.8));
#7120=CARTESIAN_POINT('Origin',(2.5,-3.5,1.9));
#7121=CARTESIAN_POINT('',(2.225,-3.5,2.));
#7122=CARTESIAN_POINT('Origin',(2.5,-3.5,2.));
#7123=CARTESIAN_POINT('',(2.225,-3.5,2.8));
#7124=CARTESIAN_POINT('',(2.225,-3.5,1.9));
#7125=CARTESIAN_POINT('Origin',(2.5,-3.5,2.8));
#7126=CARTESIAN_POINT('Origin',(19.5,3.5,1.9));
#7127=CARTESIAN_POINT('',(19.225,3.5,2.));
#7128=CARTESIAN_POINT('Origin',(19.5,3.5,2.));
#7129=CARTESIAN_POINT('',(19.225,3.5,2.8));
#7130=CARTESIAN_POINT('',(19.225,3.5,1.9));
#7131=CARTESIAN_POINT('Origin',(19.5,3.5,2.8));
#7132=CARTESIAN_POINT('Origin',(14.,0.,1.9));
#7133=CARTESIAN_POINT('',(13.835,-2.02066721859312E-17,2.));
#7134=CARTESIAN_POINT('Origin',(14.,0.,2.));
#7135=CARTESIAN_POINT('',(13.835,2.02066721859312E-17,2.8));
#7136=CARTESIAN_POINT('',(13.835,-2.02066721859312E-17,1.9));
#7137=CARTESIAN_POINT('Origin',(14.,0.,2.8));
#7138=CARTESIAN_POINT('Origin',(8.,0.,1.9));
#7139=CARTESIAN_POINT('',(7.835,-2.02066721859312E-17,2.));
#7140=CARTESIAN_POINT('Origin',(8.,0.,2.));
#7141=CARTESIAN_POINT('',(7.835,2.02066721859312E-17,2.8));
#7142=CARTESIAN_POINT('',(7.835,-2.02066721859312E-17,1.9));
#7143=CARTESIAN_POINT('Origin',(8.,0.,2.8));
#7144=CARTESIAN_POINT('Origin',(2.,0.,1.9));
#7145=CARTESIAN_POINT('',(1.835,-2.02066721859313E-17,2.));
#7146=CARTESIAN_POINT('Origin',(2.,0.,2.));
#7147=CARTESIAN_POINT('',(1.835,2.02066721859313E-17,2.8));
#7148=CARTESIAN_POINT('',(1.835,-2.02066721859313E-17,1.9));
#7149=CARTESIAN_POINT('Origin',(2.,0.,2.8));
#7150=CARTESIAN_POINT('Origin',(20.,0.,1.9));
#7151=CARTESIAN_POINT('',(19.835,-2.02066721859312E-17,2.));
#7152=CARTESIAN_POINT('Origin',(20.,0.,2.));
#7153=CARTESIAN_POINT('',(19.835,2.02066721859312E-17,2.8));
#7154=CARTESIAN_POINT('',(19.835,-2.02066721859312E-17,1.9));
#7155=CARTESIAN_POINT('Origin',(20.,0.,2.8));
#7156=CARTESIAN_POINT('Origin',(24.,5.,2.));
#7157=CARTESIAN_POINT('',(24.,5.,2.));
#7158=CARTESIAN_POINT('',(-2.,5.,2.));
#7159=CARTESIAN_POINT('',(24.,5.,2.));
#7160=CARTESIAN_POINT('',(-2.,5.,2.8));
#7161=CARTESIAN_POINT('',(-2.,5.,2.));
#7162=CARTESIAN_POINT('',(24.,5.,2.8));
#7163=CARTESIAN_POINT('',(24.,5.,2.8));
#7164=CARTESIAN_POINT('',(24.,5.,2.));
#7165=CARTESIAN_POINT('Origin',(24.,-5.,2.));
#7166=CARTESIAN_POINT('',(24.,-5.,2.));
#7167=CARTESIAN_POINT('',(24.,-5.,2.));
#7168=CARTESIAN_POINT('',(24.,-5.,2.8));
#7169=CARTESIAN_POINT('',(24.,-5.,2.8));
#7170=CARTESIAN_POINT('',(24.,-5.,2.));
#7171=CARTESIAN_POINT('Origin',(-2.,-5.,2.));
#7172=CARTESIAN_POINT('',(-2.,-5.,2.));
#7173=CARTESIAN_POINT('',(-2.,-5.,2.));
#7174=CARTESIAN_POINT('',(-2.,-5.,2.8));
#7175=CARTESIAN_POINT('',(-2.,-5.,2.8));
#7176=CARTESIAN_POINT('',(-2.,-5.,2.));
#7177=CARTESIAN_POINT('Origin',(-2.,5.,2.));
#7178=CARTESIAN_POINT('',(-2.,5.,2.));
#7179=CARTESIAN_POINT('',(-2.,5.,2.8));
#7180=CARTESIAN_POINT('Origin',(11.,0.,2.8));
#7181=CARTESIAN_POINT('Origin',(11.,0.,2.));
#8456=UNCERTAINTY_MEASURE_WITH_UNIT(LENGTH_MEASURE(0.001),#8500,
'DISTANCE_ACCURACY_VALUE',
'Maximum model space distance between geometric entities at asserted c
onnectivities');
#8476=UNCERTAINTY_MEASURE_WITH_UNIT(LENGTH_MEASURE(0.001),#8500,
'DISTANCE_ACCURACY_VALUE',
'Maximum model space distance between geometric entities at asserted c
onnectivities');
#8479=(
GEOMETRIC_REPRESENTATION_CONTEXT(3)
GLOBAL_UNCERTAINTY_ASSIGNED_CONTEXT((#8456))
GLOBAL_UNIT_ASSIGNED_CONTEXT((#8500,#8502,#8503))
REPRESENTATION_CONTEXT('','3D')
);
#8499=(
GEOMETRIC_REPRESENTATION_CONTEXT(3)
GLOBAL_UNCERTAINTY_ASSIGNED_CONTEXT((#8476))
GLOBAL_UNIT_ASSIGNED_CONTEXT((#8500,#8502,#8503))
REPRESENTATION_CONTEXT('','3D')
);
#8500=(
LENGTH_UNIT()
NAMED_UNIT(*)
SI_UNIT(.CENTI.,.METRE.)
);
#8502=(
NAMED_UNIT(*)
PLANE_ANGLE_UNIT()
SI_UNIT($,.RADIAN.)
);
#8503=(
NAMED_UNIT(*)
SI_UNIT($,.STERADIAN.)
SOLID_ANGLE_UNIT()
);
#8506=SHAPE_DEFINITION_REPRESENTATION(#8528,#8600);
#8528=PRODUCT_DEFINITION_SHAPE('',$,#8623);
#8600=SHAPE_REPRESENTATION('',(#5164),#8479);
#8620=PRODUCT_DEFINITION_CONTEXT('part definition',#8688,'design');
#8623=PRODUCT_DEFINITION('Base plate','Base plate',#8645,#8620);
#8645=PRODUCT_DEFINITION_FORMATION('',$,#8692);
#8688=APPLICATION_CONTEXT(
'Core Data for Automotive Mechanical Design Process');
#8689=PRODUCT_CONTEXT('part definition',#8688,'mechanical');
#8692=PRODUCT('Base plate','Base plate','Base plate',(#8689));
#8761=COLOUR_RGB('Dark Blue',0.08,0.2,0.34);
#8762=FILL_AREA_STYLE_COLOUR('',#8761);
#8763=FILL_AREA_STYLE('',(#8762));
#8764=SURFACE_STYLE_FILL_AREA(#8763);
#8765=SURFACE_SIDE_STYLE('',(#8764));
#8766=SURFACE_STYLE_USAGE(.BOTH.,#8765);
#8767=PRESENTATION_STYLE_ASSIGNMENT((#8766));
ENDSEC;
END-ISO-10303-21;
